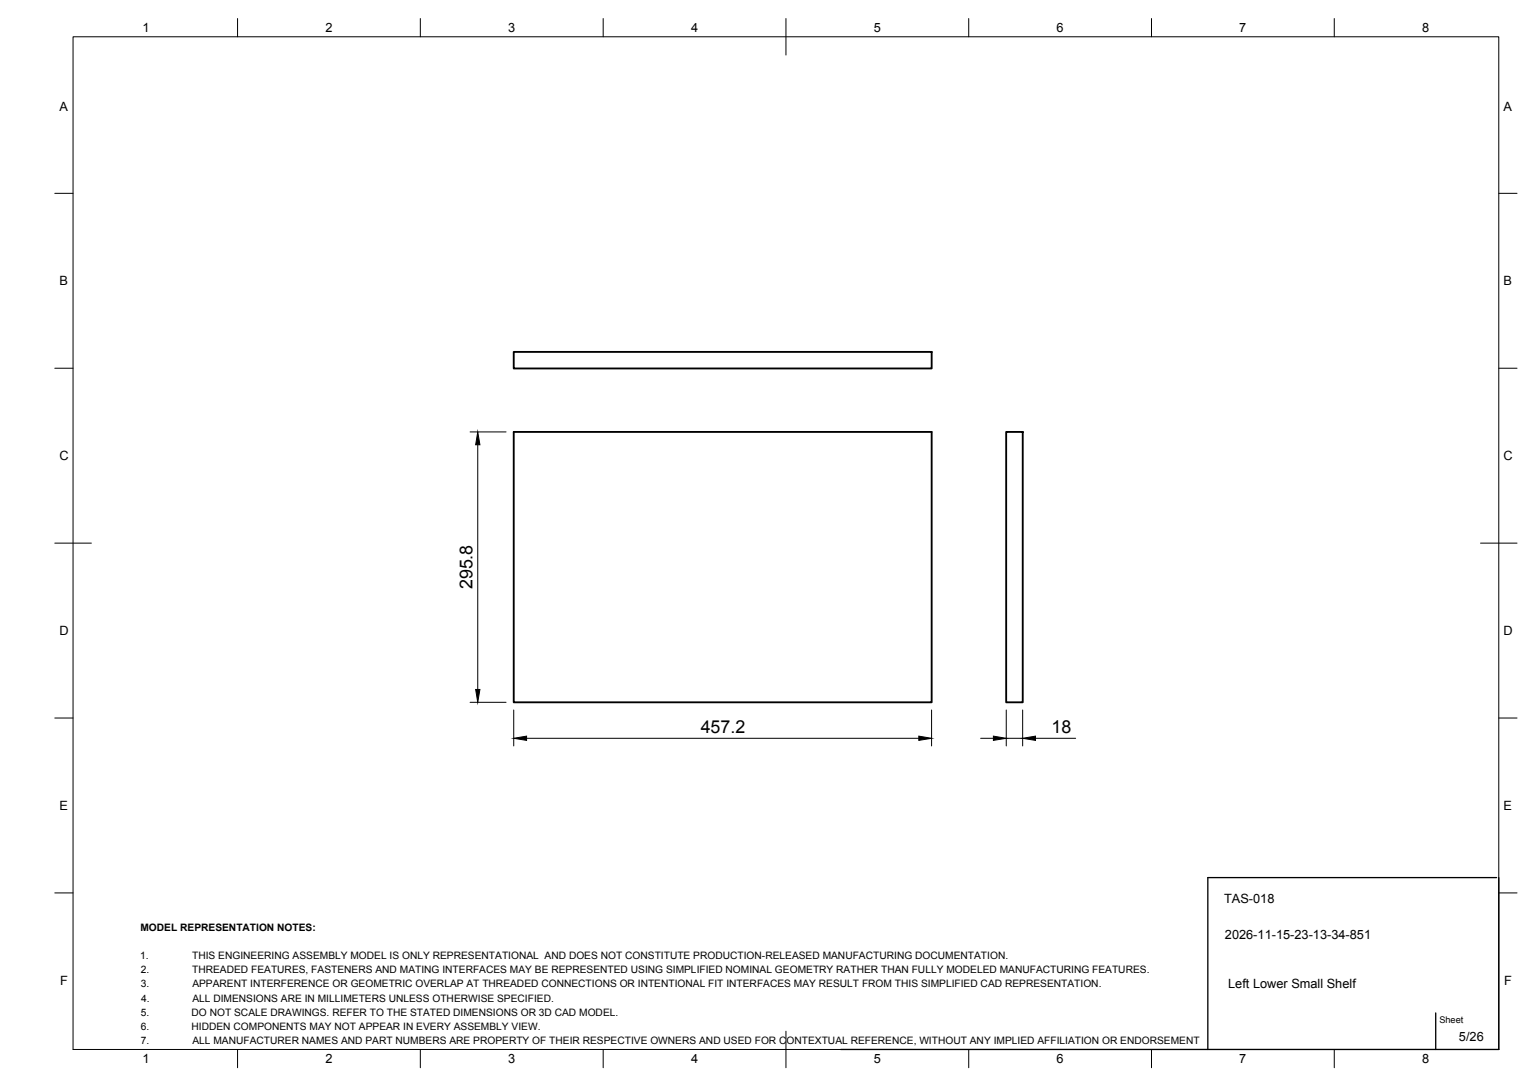
ISO-10303-21;
HEADER;
/* Generated by software containing ST-Developer
 * from STEP Tools, Inc. (www.steptools.com) 
 */

FILE_DESCRIPTION(
/* description */ (''),
/* implementation_level */ '2;1');

FILE_NAME(
/* name */ 'Left Lower Small Shelf.step',
/* time_stamp */ '2026-11-15T15:17:57-08:00',
/* author */ (''),
/* organization */ (''),
/* preprocessor_version */ 'ST-DEVELOPER v20.2',
/* originating_system */ 'Autodesk Translation Framework v15.17.0.0',
/* authorisation */ '');

FILE_SCHEMA (('AUTOMOTIVE_DESIGN { 1 0 10303 214 3 1 1 }'));
ENDSEC;

DATA;
#10=MECHANICAL_DESIGN_GEOMETRIC_PRESENTATION_REPRESENTATION('',(#180),#3723);
#132=SHAPE_REPRESENTATION_RELATIONSHIP('SRR','None',#3813,#156);
#156=ADVANCED_BREP_SHAPE_REPRESENTATION('',(#204),#3702);
#180=STYLED_ITEM('',(#3944),#204);
#204=MANIFOLD_SOLID_BREP('Body1',#2028);
#243=FACE_OUTER_BOUND('',#369,.T.);
#244=FACE_OUTER_BOUND('',#370,.T.);
#245=FACE_OUTER_BOUND('',#371,.T.);
#246=FACE_OUTER_BOUND('',#372,.T.);
#247=FACE_OUTER_BOUND('',#373,.T.);
#248=FACE_OUTER_BOUND('',#374,.T.);
#369=EDGE_LOOP('',(#1383,#1384,#1385,#1386));
#370=EDGE_LOOP('',(#1387,#1388,#1389,#1390));
#371=EDGE_LOOP('',(#1391,#1392,#1393,#1394));
#372=EDGE_LOOP('',(#1395,#1396,#1397,#1398));
#373=EDGE_LOOP('',(#1399,#1400,#1401,#1402));
#374=EDGE_LOOP('',(#1403,#1404,#1405,#1406));
#513=LINE('',#3191,#735);
#514=LINE('',#3193,#736);
#515=LINE('',#3195,#737);
#516=LINE('',#3196,#738);
#517=LINE('',#3199,#739);
#518=LINE('',#3201,#740);
#519=LINE('',#3202,#741);
#520=LINE('',#3205,#742);
#521=LINE('',#3207,#743);
#522=LINE('',#3208,#744);
#523=LINE('',#3210,#745);
#524=LINE('',#3211,#746);
#735=VECTOR('',#2591,0.708661417322833);
#736=VECTOR('',#2592,18.);
#737=VECTOR('',#2593,0.708661417322833);
#738=VECTOR('',#2594,18.);
#739=VECTOR('',#2597,11.6456692913385);
#740=VECTOR('',#2598,11.6456692913385);
#741=VECTOR('',#2599,18.);
#742=VECTOR('',#2602,0.708661417322833);
#743=VECTOR('',#2603,0.708661417322833);
#744=VECTOR('',#2604,18.);
#745=VECTOR('',#2607,11.6456692913385);
#746=VECTOR('',#2608,11.6456692913385);
#945=VERTEX_POINT('',#3189);
#946=VERTEX_POINT('',#3190);
#947=VERTEX_POINT('',#3192);
#948=VERTEX_POINT('',#3194);
#949=VERTEX_POINT('',#3198);
#950=VERTEX_POINT('',#3200);
#951=VERTEX_POINT('',#3204);
#952=VERTEX_POINT('',#3206);
#1113=EDGE_CURVE('',#945,#946,#513,.T.);
#1114=EDGE_CURVE('',#945,#947,#514,.T.);
#1115=EDGE_CURVE('',#947,#948,#515,.T.);
#1116=EDGE_CURVE('',#946,#948,#516,.T.);
#1117=EDGE_CURVE('',#946,#949,#517,.T.);
#1118=EDGE_CURVE('',#948,#950,#518,.T.);
#1119=EDGE_CURVE('',#949,#950,#519,.T.);
#1120=EDGE_CURVE('',#949,#951,#520,.T.);
#1121=EDGE_CURVE('',#950,#952,#521,.T.);
#1122=EDGE_CURVE('',#951,#952,#522,.T.);
#1123=EDGE_CURVE('',#951,#945,#523,.T.);
#1124=EDGE_CURVE('',#952,#947,#524,.T.);
#1383=ORIENTED_EDGE('',*,*,#1113,.F.);
#1384=ORIENTED_EDGE('',*,*,#1114,.T.);
#1385=ORIENTED_EDGE('',*,*,#1115,.T.);
#1386=ORIENTED_EDGE('',*,*,#1116,.F.);
#1387=ORIENTED_EDGE('',*,*,#1117,.F.);
#1388=ORIENTED_EDGE('',*,*,#1116,.T.);
#1389=ORIENTED_EDGE('',*,*,#1118,.T.);
#1390=ORIENTED_EDGE('',*,*,#1119,.F.);
#1391=ORIENTED_EDGE('',*,*,#1120,.F.);
#1392=ORIENTED_EDGE('',*,*,#1119,.T.);
#1393=ORIENTED_EDGE('',*,*,#1121,.T.);
#1394=ORIENTED_EDGE('',*,*,#1122,.F.);
#1395=ORIENTED_EDGE('',*,*,#1123,.F.);
#1396=ORIENTED_EDGE('',*,*,#1122,.T.);
#1397=ORIENTED_EDGE('',*,*,#1124,.T.);
#1398=ORIENTED_EDGE('',*,*,#1114,.F.);
#1399=ORIENTED_EDGE('',*,*,#1115,.F.);
#1400=ORIENTED_EDGE('',*,*,#1124,.F.);
#1401=ORIENTED_EDGE('',*,*,#1121,.F.);
#1402=ORIENTED_EDGE('',*,*,#1118,.F.);
#1403=ORIENTED_EDGE('',*,*,#1123,.T.);
#1404=ORIENTED_EDGE('',*,*,#1113,.T.);
#1405=ORIENTED_EDGE('',*,*,#1117,.T.);
#1406=ORIENTED_EDGE('',*,*,#1120,.T.);
#1797=PLANE('',#2339);
#1798=PLANE('',#2340);
#1799=PLANE('',#2341);
#1800=PLANE('',#2342);
#1801=PLANE('',#2343);
#1802=PLANE('',#2344);
#1917=ADVANCED_FACE('',(#243),#1797,.F.);
#1918=ADVANCED_FACE('',(#244),#1798,.F.);
#1919=ADVANCED_FACE('',(#245),#1799,.F.);
#1920=ADVANCED_FACE('',(#246),#1800,.F.);
#1921=ADVANCED_FACE('',(#247),#1801,.F.);
#1922=ADVANCED_FACE('',(#248),#1802,.T.);
#2028=CLOSED_SHELL('',(#1917,#1918,#1919,#1920,#1921,#1922));
#2338=AXIS2_PLACEMENT_3D('',#3187,#2587,#2588);
#2339=AXIS2_PLACEMENT_3D('',#3188,#2589,#2590);
#2340=AXIS2_PLACEMENT_3D('',#3197,#2595,#2596);
#2341=AXIS2_PLACEMENT_3D('',#3203,#2600,#2601);
#2342=AXIS2_PLACEMENT_3D('',#3209,#2605,#2606);
#2343=AXIS2_PLACEMENT_3D('',#3212,#2609,#2610);
#2344=AXIS2_PLACEMENT_3D('',#3213,#2611,#2612);
#2587=DIRECTION('axis',(0.,0.,1.));
#2588=DIRECTION('refdir',(1.,0.,0.));
#2589=DIRECTION('center_axis',(-1.,0.,0.));
#2590=DIRECTION('ref_axis',(0.,0.,1.));
#2591=DIRECTION('',(0.,1.,0.));
#2592=DIRECTION('',(0.,0.,-1.));
#2593=DIRECTION('',(0.,1.,0.));
#2594=DIRECTION('',(0.,0.,-1.));
#2595=DIRECTION('center_axis',(0.,-1.,0.));
#2596=DIRECTION('ref_axis',(0.,0.,-1.));
#2597=DIRECTION('',(-1.,0.,0.));
#2598=DIRECTION('',(-1.,0.,0.));
#2599=DIRECTION('',(0.,0.,-1.));
#2600=DIRECTION('center_axis',(1.,0.,0.));
#2601=DIRECTION('ref_axis',(0.,0.,-1.));
#2602=DIRECTION('',(0.,-1.,0.));
#2603=DIRECTION('',(0.,-1.,0.));
#2604=DIRECTION('',(0.,0.,-1.));
#2605=DIRECTION('center_axis',(0.,1.,0.));
#2606=DIRECTION('ref_axis',(0.,0.,1.));
#2607=DIRECTION('',(1.,0.,0.));
#2608=DIRECTION('',(1.,0.,0.));
#2609=DIRECTION('center_axis',(0.,0.,1.));
#2610=DIRECTION('ref_axis',(1.,0.,0.));
#2611=DIRECTION('center_axis',(0.,0.,1.));
#2612=DIRECTION('ref_axis',(1.,0.,0.));
#3187=CARTESIAN_POINT('',(0.,0.,0.));
#3188=CARTESIAN_POINT('Origin',(-0.354330708661442,39.3359580052493,30.375872491424));
#3189=CARTESIAN_POINT('',(-0.354330708661442,38.6272965879265,18.7086614173228));
#3190=CARTESIAN_POINT('',(-0.354330708661442,39.3359580052493,18.7086614173228));
#3191=CARTESIAN_POINT('',(-0.354330708661442,38.6272965879265,18.7086614173228));
#3192=CARTESIAN_POINT('',(-0.354330708661442,38.6272965879265,0.708661417322834));
#3193=CARTESIAN_POINT('',(-0.354330708661442,38.6272965879265,18.7086614173228));
#3194=CARTESIAN_POINT('',(-0.354330708661442,39.3359580052493,0.708661417322834));
#3195=CARTESIAN_POINT('',(-0.354330708661442,38.6272965879265,0.708661417322834));
#3196=CARTESIAN_POINT('',(-0.354330708661442,39.3359580052493,18.7086614173228));
#3197=CARTESIAN_POINT('Origin',(-12.,39.3359580052493,30.375872491424));
#3198=CARTESIAN_POINT('',(-12.,39.3359580052493,18.7086614173228));
#3199=CARTESIAN_POINT('',(-0.354330708661442,39.3359580052493,18.7086614173228));
#3200=CARTESIAN_POINT('',(-12.,39.3359580052493,0.708661417322834));
#3201=CARTESIAN_POINT('',(-0.354330708661446,39.3359580052493,0.708661417322834));
#3202=CARTESIAN_POINT('',(-12.,39.3359580052493,18.7086614173228));
#3203=CARTESIAN_POINT('Origin',(-12.,39.3359580052493,30.375872491424));
#3204=CARTESIAN_POINT('',(-12.,38.6272965879265,18.7086614173228));
#3205=CARTESIAN_POINT('',(-12.,39.3359580052493,18.7086614173228));
#3206=CARTESIAN_POINT('',(-12.,38.6272965879265,0.708661417322834));
#3207=CARTESIAN_POINT('',(-12.,39.3359580052493,0.708661417322834));
#3208=CARTESIAN_POINT('',(-12.,38.6272965879265,18.7086614173228));
#3209=CARTESIAN_POINT('Origin',(-12.,38.6272965879265,30.375872491424));
#3210=CARTESIAN_POINT('',(-12.,38.6272965879265,18.7086614173228));
#3211=CARTESIAN_POINT('',(-12.,38.6272965879265,0.708661417322834));
#3212=CARTESIAN_POINT('Origin',(0.,0.,0.708661417322834));
#3213=CARTESIAN_POINT('Origin',(0.,0.,18.7086614173228));
#3675=UNCERTAINTY_MEASURE_WITH_UNIT(LENGTH_MEASURE(0.000393700787401575),
#3725,'DISTANCE_ACCURACY_VALUE',
'Maximum model space distance between geometric entities at asserted c
onnectivities');
#3696=UNCERTAINTY_MEASURE_WITH_UNIT(LENGTH_MEASURE(0.000393700787401575),
#3725,'DISTANCE_ACCURACY_VALUE',
'Maximum model space distance between geometric entities at asserted c
onnectivities');
#3702=(
GEOMETRIC_REPRESENTATION_CONTEXT(3)
GLOBAL_UNCERTAINTY_ASSIGNED_CONTEXT((#3675))
GLOBAL_UNIT_ASSIGNED_CONTEXT((#3725,#3729,#3730))
REPRESENTATION_CONTEXT('','3D')
);
#3723=(
GEOMETRIC_REPRESENTATION_CONTEXT(3)
GLOBAL_UNCERTAINTY_ASSIGNED_CONTEXT((#3696))
GLOBAL_UNIT_ASSIGNED_CONTEXT((#3725,#3729,#3730))
REPRESENTATION_CONTEXT('','3D')
);
#3724=DIMENSIONAL_EXPONENTS(1.,0.,0.,0.,0.,0.,0.);
#3725=(
CONVERSION_BASED_UNIT('inch',#3728)
LENGTH_UNIT()
NAMED_UNIT(#3724)
);
#3726=(
LENGTH_UNIT()
NAMED_UNIT(*)
SI_UNIT(.MILLI.,.METRE.)
);
#3728=LENGTH_MEASURE_WITH_UNIT(LENGTH_MEASURE(25.4),#3726);
#3729=(
NAMED_UNIT(*)
PLANE_ANGLE_UNIT()
SI_UNIT($,.RADIAN.)
);
#3730=(
NAMED_UNIT(*)
SI_UNIT($,.STERADIAN.)
SOLID_ANGLE_UNIT()
);
#3736=SHAPE_DEFINITION_REPRESENTATION(#3763,#3813);
#3763=PRODUCT_DEFINITION_SHAPE('',$,#3840);
#3813=SHAPE_REPRESENTATION('',(#2338),#3702);
#3834=PRODUCT_DEFINITION_CONTEXT('part definition',#3914,'design');
#3840=PRODUCT_DEFINITION('2026-11-15-23-13-34-851',
'Left Lower Small Shelf',#3866,#3834);
#3866=PRODUCT_DEFINITION_FORMATION('',$,#3921);
#3914=APPLICATION_CONTEXT(
'Core Data for Automotive Mechanical Design Process');
#3915=PRODUCT_CONTEXT('part definition',#3914,'mechanical');
#3921=PRODUCT('2026-11-15-23-13-34-851','Left Lower Small Shelf',$,(#3915));
#3944=PRESENTATION_STYLE_ASSIGNMENT((#3952));
#3952=SURFACE_STYLE_USAGE(.BOTH.,#3960);
#3960=SURFACE_SIDE_STYLE('',(#3968));
#3968=SURFACE_STYLE_FILL_AREA(#3976);
#3976=FILL_AREA_STYLE('Light Gray',(#3984));
#3984=FILL_AREA_STYLE_COLOUR('Light Gray',#3992);
#3992=COLOUR_RGB('Light Gray',0.827450980392157,0.827450980392157,0.827450980392157);
ENDSEC;
END-ISO-10303-21;
